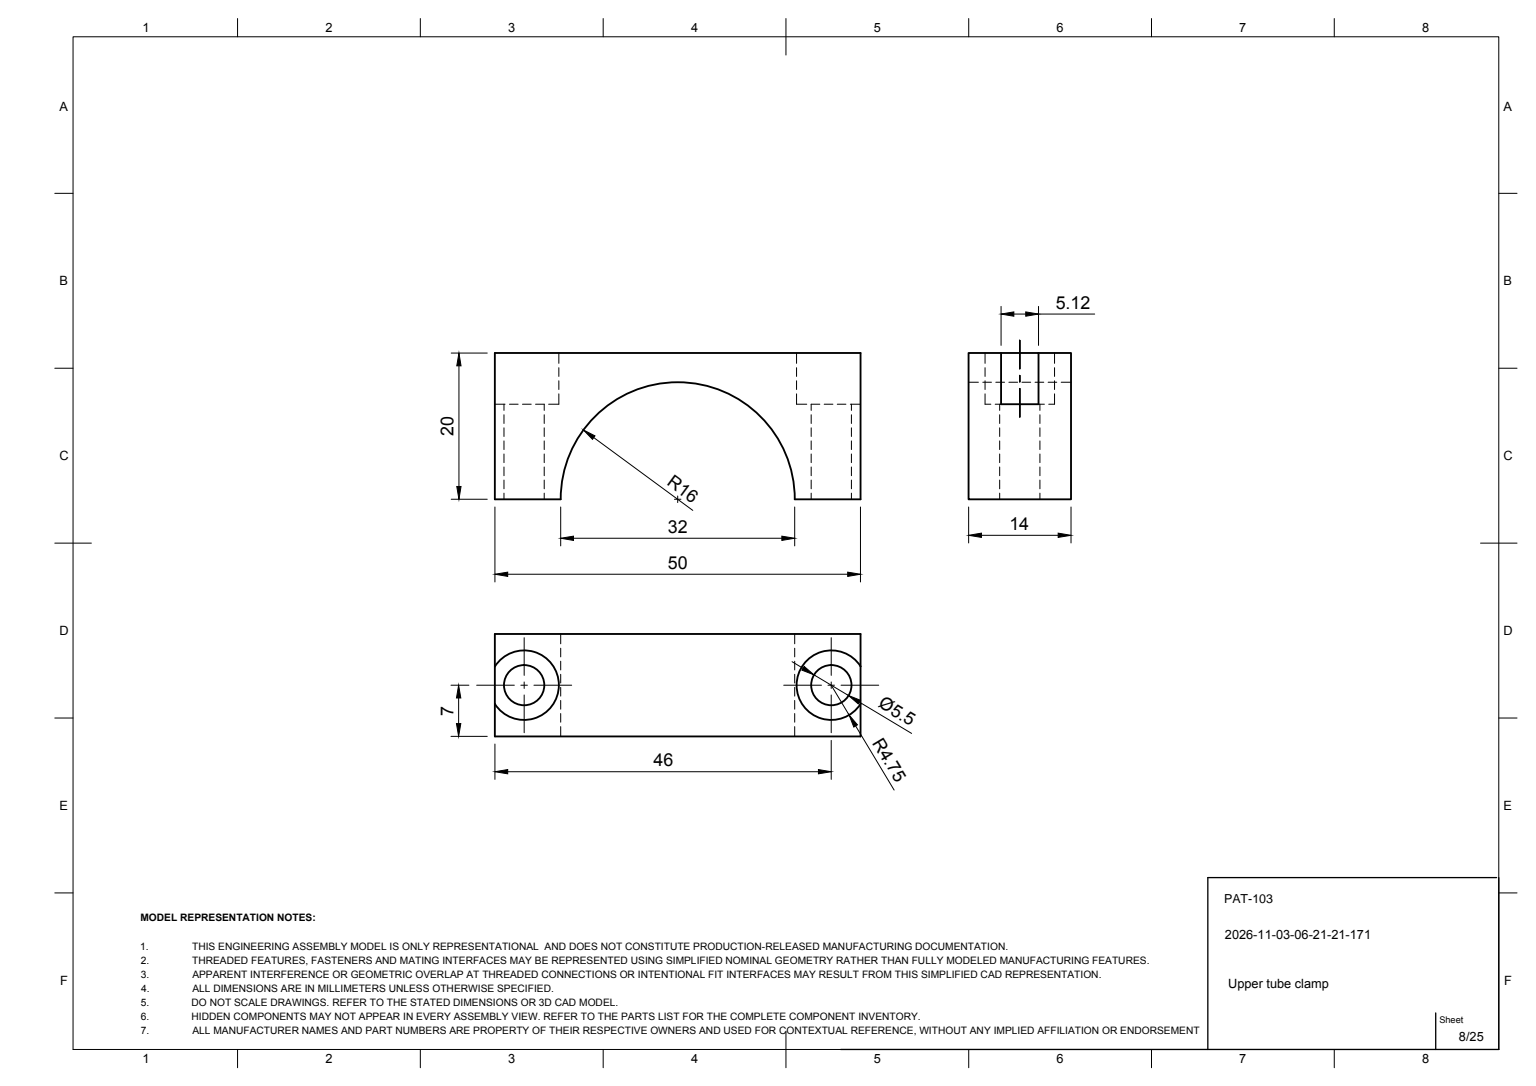
ISO-10303-21;
HEADER;
/* Generated by software containing ST-Developer
 * from STEP Tools, Inc. (www.steptools.com) 
 */

FILE_DESCRIPTION(
/* description */ ('Telescoping shaft support with lock collar'),
/* implementation_level */ '2;1');

FILE_NAME(
/* name */ 'Upper tube clamp.step',
/* time_stamp */ '2026-10-27T10:48:51-07:00',
/* author */ (''),
/* organization */ (''),
/* preprocessor_version */ 'ST-DEVELOPER v20.2',
/* originating_system */ 'Autodesk Translation Framework v15.17.0.0',
/* authorisation */ '');

FILE_SCHEMA (('AUTOMOTIVE_DESIGN { 1 0 10303 214 3 1 1 }'));
ENDSEC;

DATA;
#10=MECHANICAL_DESIGN_GEOMETRIC_PRESENTATION_REPRESENTATION('',(#244),#7349);
#204=SHAPE_REPRESENTATION_RELATIONSHIP('SRR','None',#7446,#224);
#224=ADVANCED_BREP_SHAPE_REPRESENTATION('',(#264),#7330);
#244=STYLED_ITEM('',(#7641),#264);
#264=MANIFOLD_SOLID_BREP('Body1',#3967);
#301=FACE_BOUND('',#790,.T.);
#302=FACE_BOUND('',#793,.T.);
#303=FACE_BOUND('',#802,.T.);
#304=FACE_BOUND('',#806,.T.);
#386=PLANE('',#4321);
#387=PLANE('',#4326);
#388=PLANE('',#4331);
#389=PLANE('',#4332);
#390=PLANE('',#4340);
#391=PLANE('',#4341);
#392=PLANE('',#4342);
#393=PLANE('',#4343);
#394=PLANE('',#4344);
#541=FACE_OUTER_BOUND('',#789,.T.);
#542=FACE_OUTER_BOUND('',#791,.T.);
#543=FACE_OUTER_BOUND('',#792,.T.);
#544=FACE_OUTER_BOUND('',#794,.T.);
#545=FACE_OUTER_BOUND('',#795,.T.);
#546=FACE_OUTER_BOUND('',#796,.T.);
#547=FACE_OUTER_BOUND('',#797,.T.);
#548=FACE_OUTER_BOUND('',#798,.T.);
#549=FACE_OUTER_BOUND('',#799,.T.);
#550=FACE_OUTER_BOUND('',#800,.T.);
#551=FACE_OUTER_BOUND('',#801,.T.);
#552=FACE_OUTER_BOUND('',#803,.T.);
#553=FACE_OUTER_BOUND('',#804,.T.);
#554=FACE_OUTER_BOUND('',#805,.T.);
#789=EDGE_LOOP('',(#2882,#2883));
#790=EDGE_LOOP('',(#2884));
#791=EDGE_LOOP('',(#2885,#2886,#2887,#2888));
#792=EDGE_LOOP('',(#2889,#2890));
#793=EDGE_LOOP('',(#2891));
#794=EDGE_LOOP('',(#2892,#2893,#2894,#2895));
#795=EDGE_LOOP('',(#2896,#2897,#2898,#2899,#2900,#2901,#2902,#2903));
#796=EDGE_LOOP('',(#2904,#2905,#2906,#2907,#2908,#2909,#2910,#2911));
#797=EDGE_LOOP('',(#2912,#2913,#2914,#2915));
#798=EDGE_LOOP('',(#2916,#2917,#2918,#2919));
#799=EDGE_LOOP('',(#2920,#2921,#2922,#2923));
#800=EDGE_LOOP('',(#2924,#2925,#2926,#2927,#2928,#2929));
#801=EDGE_LOOP('',(#2930,#2931,#2932,#2933));
#802=EDGE_LOOP('',(#2934));
#803=EDGE_LOOP('',(#2935,#2936,#2937,#2938,#2939,#2940));
#804=EDGE_LOOP('',(#2941,#2942,#2943,#2944,#2945,#2946,#2947,#2948));
#805=EDGE_LOOP('',(#2949,#2950,#2951,#2952));
#806=EDGE_LOOP('',(#2953));
#1085=LINE('',#6242,#1365);
#1086=LINE('',#6248,#1366);
#1087=LINE('',#6251,#1367);
#1088=LINE('',#6255,#1368);
#1089=LINE('',#6261,#1369);
#1090=LINE('',#6264,#1370);
#1091=LINE('',#6267,#1371);
#1092=LINE('',#6269,#1372);
#1093=LINE('',#6271,#1373);
#1094=LINE('',#6273,#1374);
#1095=LINE('',#6274,#1375);
#1096=LINE('',#6277,#1376);
#1097=LINE('',#6279,#1377);
#1098=LINE('',#6281,#1378);
#1099=LINE('',#6283,#1379);
#1100=LINE('',#6284,#1380);
#1101=LINE('',#6288,#1381);
#1102=LINE('',#6292,#1382);
#1103=LINE('',#6298,#1383);
#1104=LINE('',#6301,#1384);
#1105=LINE('',#6303,#1385);
#1106=LINE('',#6304,#1386);
#1107=LINE('',#6305,#1387);
#1108=LINE('',#6307,#1388);
#1109=LINE('',#6309,#1389);
#1110=LINE('',#6310,#1390);
#1365=VECTOR('',#4995,1.);
#1366=VECTOR('',#5002,1.);
#1367=VECTOR('',#5005,1.);
#1368=VECTOR('',#5008,1.);
#1369=VECTOR('',#5015,1.);
#1370=VECTOR('',#5018,1.);
#1371=VECTOR('',#5021,1.);
#1372=VECTOR('',#5022,1.);
#1373=VECTOR('',#5023,1.);
#1374=VECTOR('',#5024,1.);
#1375=VECTOR('',#5025,1.);
#1376=VECTOR('',#5028,1.);
#1377=VECTOR('',#5029,1.);
#1378=VECTOR('',#5030,1.);
#1379=VECTOR('',#5031,1.);
#1380=VECTOR('',#5032,1.);
#1381=VECTOR('',#5037,0.275);
#1382=VECTOR('',#5042,0.275);
#1383=VECTOR('',#5047,1.);
#1384=VECTOR('',#5050,1.);
#1385=VECTOR('',#5053,1.);
#1386=VECTOR('',#5054,1.);
#1387=VECTOR('',#5055,1.);
#1388=VECTOR('',#5058,1.);
#1389=VECTOR('',#5061,1.);
#1390=VECTOR('',#5062,1.);
#1649=CIRCLE('',#4322,0.475);
#1650=CIRCLE('',#4323,0.275);
#1651=CIRCLE('',#4325,0.475);
#1652=CIRCLE('',#4327,0.475);
#1653=CIRCLE('',#4328,0.275);
#1654=CIRCLE('',#4330,0.475);
#1655=CIRCLE('',#4334,0.275);
#1656=CIRCLE('',#4336,0.275);
#1657=CIRCLE('',#4338,1.6);
#1658=CIRCLE('',#4339,1.6);
#1878=VERTEX_POINT('',#6240);
#1879=VERTEX_POINT('',#6241);
#1880=VERTEX_POINT('',#6244);
#1881=VERTEX_POINT('',#6247);
#1882=VERTEX_POINT('',#6249);
#1883=VERTEX_POINT('',#6253);
#1884=VERTEX_POINT('',#6254);
#1885=VERTEX_POINT('',#6257);
#1886=VERTEX_POINT('',#6260);
#1887=VERTEX_POINT('',#6262);
#1888=VERTEX_POINT('',#6266);
#1889=VERTEX_POINT('',#6268);
#1890=VERTEX_POINT('',#6270);
#1891=VERTEX_POINT('',#6272);
#1892=VERTEX_POINT('',#6276);
#1893=VERTEX_POINT('',#6278);
#1894=VERTEX_POINT('',#6280);
#1895=VERTEX_POINT('',#6282);
#1896=VERTEX_POINT('',#6286);
#1897=VERTEX_POINT('',#6290);
#1898=VERTEX_POINT('',#6294);
#1899=VERTEX_POINT('',#6295);
#1900=VERTEX_POINT('',#6297);
#1901=VERTEX_POINT('',#6299);
#2253=EDGE_CURVE('',#1878,#1879,#1085,.T.);
#2254=EDGE_CURVE('',#1878,#1879,#1649,.T.);
#2255=EDGE_CURVE('',#1880,#1880,#1650,.T.);
#2256=EDGE_CURVE('',#1881,#1878,#1086,.T.);
#2257=EDGE_CURVE('',#1882,#1881,#1651,.T.);
#2258=EDGE_CURVE('',#1879,#1882,#1087,.T.);
#2259=EDGE_CURVE('',#1883,#1884,#1088,.T.);
#2260=EDGE_CURVE('',#1883,#1884,#1652,.T.);
#2261=EDGE_CURVE('',#1885,#1885,#1653,.T.);
#2262=EDGE_CURVE('',#1886,#1883,#1089,.T.);
#2263=EDGE_CURVE('',#1887,#1886,#1654,.T.);
#2264=EDGE_CURVE('',#1884,#1887,#1090,.T.);
#2265=EDGE_CURVE('',#1888,#1882,#1091,.T.);
#2266=EDGE_CURVE('',#1889,#1888,#1092,.T.);
#2267=EDGE_CURVE('',#1889,#1890,#1093,.T.);
#2268=EDGE_CURVE('',#1890,#1891,#1094,.T.);
#2269=EDGE_CURVE('',#1881,#1891,#1095,.T.);
#2270=EDGE_CURVE('',#1892,#1887,#1096,.T.);
#2271=EDGE_CURVE('',#1893,#1892,#1097,.T.);
#2272=EDGE_CURVE('',#1893,#1894,#1098,.T.);
#2273=EDGE_CURVE('',#1894,#1895,#1099,.T.);
#2274=EDGE_CURVE('',#1886,#1895,#1100,.T.);
#2275=EDGE_CURVE('',#1896,#1896,#1655,.T.);
#2276=EDGE_CURVE('',#1896,#1880,#1101,.T.);
#2277=EDGE_CURVE('',#1897,#1897,#1656,.T.);
#2278=EDGE_CURVE('',#1897,#1885,#1102,.T.);
#2279=EDGE_CURVE('',#1898,#1899,#1657,.T.);
#2280=EDGE_CURVE('',#1900,#1898,#1103,.T.);
#2281=EDGE_CURVE('',#1901,#1900,#1658,.T.);
#2282=EDGE_CURVE('',#1899,#1901,#1104,.T.);
#2283=EDGE_CURVE('',#1900,#1893,#1105,.T.);
#2284=EDGE_CURVE('',#1891,#1892,#1106,.T.);
#2285=EDGE_CURVE('',#1890,#1901,#1107,.T.);
#2286=EDGE_CURVE('',#1894,#1898,#1108,.T.);
#2287=EDGE_CURVE('',#1899,#1889,#1109,.T.);
#2288=EDGE_CURVE('',#1895,#1888,#1110,.T.);
#2882=ORIENTED_EDGE('',*,*,#2253,.F.);
#2883=ORIENTED_EDGE('',*,*,#2254,.T.);
#2884=ORIENTED_EDGE('',*,*,#2255,.F.);
#2885=ORIENTED_EDGE('',*,*,#2256,.F.);
#2886=ORIENTED_EDGE('',*,*,#2257,.F.);
#2887=ORIENTED_EDGE('',*,*,#2258,.F.);
#2888=ORIENTED_EDGE('',*,*,#2254,.F.);
#2889=ORIENTED_EDGE('',*,*,#2259,.F.);
#2890=ORIENTED_EDGE('',*,*,#2260,.T.);
#2891=ORIENTED_EDGE('',*,*,#2261,.F.);
#2892=ORIENTED_EDGE('',*,*,#2262,.F.);
#2893=ORIENTED_EDGE('',*,*,#2263,.F.);
#2894=ORIENTED_EDGE('',*,*,#2264,.F.);
#2895=ORIENTED_EDGE('',*,*,#2260,.F.);
#2896=ORIENTED_EDGE('',*,*,#2256,.T.);
#2897=ORIENTED_EDGE('',*,*,#2253,.T.);
#2898=ORIENTED_EDGE('',*,*,#2258,.T.);
#2899=ORIENTED_EDGE('',*,*,#2265,.F.);
#2900=ORIENTED_EDGE('',*,*,#2266,.F.);
#2901=ORIENTED_EDGE('',*,*,#2267,.T.);
#2902=ORIENTED_EDGE('',*,*,#2268,.T.);
#2903=ORIENTED_EDGE('',*,*,#2269,.F.);
#2904=ORIENTED_EDGE('',*,*,#2262,.T.);
#2905=ORIENTED_EDGE('',*,*,#2259,.T.);
#2906=ORIENTED_EDGE('',*,*,#2264,.T.);
#2907=ORIENTED_EDGE('',*,*,#2270,.F.);
#2908=ORIENTED_EDGE('',*,*,#2271,.F.);
#2909=ORIENTED_EDGE('',*,*,#2272,.T.);
#2910=ORIENTED_EDGE('',*,*,#2273,.T.);
#2911=ORIENTED_EDGE('',*,*,#2274,.F.);
#2912=ORIENTED_EDGE('',*,*,#2275,.F.);
#2913=ORIENTED_EDGE('',*,*,#2276,.T.);
#2914=ORIENTED_EDGE('',*,*,#2255,.T.);
#2915=ORIENTED_EDGE('',*,*,#2276,.F.);
#2916=ORIENTED_EDGE('',*,*,#2277,.F.);
#2917=ORIENTED_EDGE('',*,*,#2278,.T.);
#2918=ORIENTED_EDGE('',*,*,#2261,.T.);
#2919=ORIENTED_EDGE('',*,*,#2278,.F.);
#2920=ORIENTED_EDGE('',*,*,#2279,.F.);
#2921=ORIENTED_EDGE('',*,*,#2280,.F.);
#2922=ORIENTED_EDGE('',*,*,#2281,.F.);
#2923=ORIENTED_EDGE('',*,*,#2282,.F.);
#2924=ORIENTED_EDGE('',*,*,#2281,.T.);
#2925=ORIENTED_EDGE('',*,*,#2283,.T.);
#2926=ORIENTED_EDGE('',*,*,#2271,.T.);
#2927=ORIENTED_EDGE('',*,*,#2284,.F.);
#2928=ORIENTED_EDGE('',*,*,#2268,.F.);
#2929=ORIENTED_EDGE('',*,*,#2285,.T.);
#2930=ORIENTED_EDGE('',*,*,#2280,.T.);
#2931=ORIENTED_EDGE('',*,*,#2286,.F.);
#2932=ORIENTED_EDGE('',*,*,#2272,.F.);
#2933=ORIENTED_EDGE('',*,*,#2283,.F.);
#2934=ORIENTED_EDGE('',*,*,#2277,.T.);
#2935=ORIENTED_EDGE('',*,*,#2279,.T.);
#2936=ORIENTED_EDGE('',*,*,#2287,.T.);
#2937=ORIENTED_EDGE('',*,*,#2266,.T.);
#2938=ORIENTED_EDGE('',*,*,#2288,.F.);
#2939=ORIENTED_EDGE('',*,*,#2273,.F.);
#2940=ORIENTED_EDGE('',*,*,#2286,.T.);
#2941=ORIENTED_EDGE('',*,*,#2257,.T.);
#2942=ORIENTED_EDGE('',*,*,#2269,.T.);
#2943=ORIENTED_EDGE('',*,*,#2284,.T.);
#2944=ORIENTED_EDGE('',*,*,#2270,.T.);
#2945=ORIENTED_EDGE('',*,*,#2263,.T.);
#2946=ORIENTED_EDGE('',*,*,#2274,.T.);
#2947=ORIENTED_EDGE('',*,*,#2288,.T.);
#2948=ORIENTED_EDGE('',*,*,#2265,.T.);
#2949=ORIENTED_EDGE('',*,*,#2282,.T.);
#2950=ORIENTED_EDGE('',*,*,#2285,.F.);
#2951=ORIENTED_EDGE('',*,*,#2267,.F.);
#2952=ORIENTED_EDGE('',*,*,#2287,.F.);
#2953=ORIENTED_EDGE('',*,*,#2275,.T.);
#3679=CYLINDRICAL_SURFACE('',#4324,0.475);
#3680=CYLINDRICAL_SURFACE('',#4329,0.475);
#3681=CYLINDRICAL_SURFACE('',#4333,0.275);
#3682=CYLINDRICAL_SURFACE('',#4335,0.275);
#3683=CYLINDRICAL_SURFACE('',#4337,1.6);
#3784=ADVANCED_FACE('',(#541,#301),#386,.T.);
#3785=ADVANCED_FACE('',(#542),#3679,.F.);
#3786=ADVANCED_FACE('',(#543,#302),#387,.T.);
#3787=ADVANCED_FACE('',(#544),#3680,.F.);
#3788=ADVANCED_FACE('',(#545),#388,.T.);
#3789=ADVANCED_FACE('',(#546),#389,.T.);
#3790=ADVANCED_FACE('',(#547),#3681,.F.);
#3791=ADVANCED_FACE('',(#548),#3682,.F.);
#3792=ADVANCED_FACE('',(#549),#3683,.F.);
#3793=ADVANCED_FACE('',(#550),#390,.T.);
#3794=ADVANCED_FACE('',(#551,#303),#391,.F.);
#3795=ADVANCED_FACE('',(#552),#392,.T.);
#3796=ADVANCED_FACE('',(#553),#393,.T.);
#3797=ADVANCED_FACE('',(#554,#304),#394,.F.);
#3967=CLOSED_SHELL('',(#3784,#3785,#3786,#3787,#3788,#3789,#3790,#3791,
#3792,#3793,#3794,#3795,#3796,#3797));
#4320=AXIS2_PLACEMENT_3D('',#6238,#4991,#4992);
#4321=AXIS2_PLACEMENT_3D('',#6239,#4993,#4994);
#4322=AXIS2_PLACEMENT_3D('',#6243,#4996,#4997);
#4323=AXIS2_PLACEMENT_3D('',#6245,#4998,#4999);
#4324=AXIS2_PLACEMENT_3D('',#6246,#5000,#5001);
#4325=AXIS2_PLACEMENT_3D('',#6250,#5003,#5004);
#4326=AXIS2_PLACEMENT_3D('',#6252,#5006,#5007);
#4327=AXIS2_PLACEMENT_3D('',#6256,#5009,#5010);
#4328=AXIS2_PLACEMENT_3D('',#6258,#5011,#5012);
#4329=AXIS2_PLACEMENT_3D('',#6259,#5013,#5014);
#4330=AXIS2_PLACEMENT_3D('',#6263,#5016,#5017);
#4331=AXIS2_PLACEMENT_3D('',#6265,#5019,#5020);
#4332=AXIS2_PLACEMENT_3D('',#6275,#5026,#5027);
#4333=AXIS2_PLACEMENT_3D('',#6285,#5033,#5034);
#4334=AXIS2_PLACEMENT_3D('',#6287,#5035,#5036);
#4335=AXIS2_PLACEMENT_3D('',#6289,#5038,#5039);
#4336=AXIS2_PLACEMENT_3D('',#6291,#5040,#5041);
#4337=AXIS2_PLACEMENT_3D('',#6293,#5043,#5044);
#4338=AXIS2_PLACEMENT_3D('',#6296,#5045,#5046);
#4339=AXIS2_PLACEMENT_3D('',#6300,#5048,#5049);
#4340=AXIS2_PLACEMENT_3D('',#6302,#5051,#5052);
#4341=AXIS2_PLACEMENT_3D('',#6306,#5056,#5057);
#4342=AXIS2_PLACEMENT_3D('',#6308,#5059,#5060);
#4343=AXIS2_PLACEMENT_3D('',#6311,#5063,#5064);
#4344=AXIS2_PLACEMENT_3D('',#6312,#5065,#5066);
#4991=DIRECTION('axis',(0.,0.,1.));
#4992=DIRECTION('refdir',(1.,0.,0.));
#4993=DIRECTION('center_axis',(0.,0.,1.));
#4994=DIRECTION('ref_axis',(1.,0.,0.));
#4995=DIRECTION('',(-1.,0.,0.));
#4996=DIRECTION('center_axis',(0.,0.,1.));
#4997=DIRECTION('ref_axis',(1.,0.,0.));
#4998=DIRECTION('center_axis',(0.,0.,1.));
#4999=DIRECTION('ref_axis',(1.,0.,0.));
#5000=DIRECTION('center_axis',(0.,0.,1.));
#5001=DIRECTION('ref_axis',(2.83276944882399E-16,1.,0.));
#5002=DIRECTION('',(0.,0.,-1.));
#5003=DIRECTION('center_axis',(0.,0.,-1.));
#5004=DIRECTION('ref_axis',(1.,0.,0.));
#5005=DIRECTION('',(0.,0.,1.));
#5006=DIRECTION('center_axis',(0.,0.,1.));
#5007=DIRECTION('ref_axis',(1.,0.,0.));
#5008=DIRECTION('',(1.,0.,0.));
#5009=DIRECTION('center_axis',(0.,0.,1.));
#5010=DIRECTION('ref_axis',(1.,0.,0.));
#5011=DIRECTION('center_axis',(0.,0.,1.));
#5012=DIRECTION('ref_axis',(1.,0.,0.));
#5013=DIRECTION('center_axis',(0.,0.,1.));
#5014=DIRECTION('ref_axis',(-1.83697019872103E-16,-1.,0.));
#5015=DIRECTION('',(0.,0.,-1.));
#5016=DIRECTION('center_axis',(0.,0.,-1.));
#5017=DIRECTION('ref_axis',(1.,0.,0.));
#5018=DIRECTION('',(0.,0.,1.));
#5019=DIRECTION('center_axis',(0.,-1.,0.));
#5020=DIRECTION('ref_axis',(1.,0.,0.));
#5021=DIRECTION('',(1.,0.,0.));
#5022=DIRECTION('',(0.,0.,1.));
#5023=DIRECTION('',(1.,0.,0.));
#5024=DIRECTION('',(0.,0.,1.));
#5025=DIRECTION('',(1.,0.,0.));
#5026=DIRECTION('center_axis',(0.,1.,0.));
#5027=DIRECTION('ref_axis',(-1.,0.,0.));
#5028=DIRECTION('',(-1.,0.,0.));
#5029=DIRECTION('',(0.,0.,1.));
#5030=DIRECTION('',(-1.,0.,0.));
#5031=DIRECTION('',(0.,0.,1.));
#5032=DIRECTION('',(-1.,0.,0.));
#5033=DIRECTION('center_axis',(0.,0.,1.));
#5034=DIRECTION('ref_axis',(1.,0.,0.));
#5035=DIRECTION('center_axis',(0.,0.,1.));
#5036=DIRECTION('ref_axis',(1.,0.,0.));
#5037=DIRECTION('',(0.,0.,1.));
#5038=DIRECTION('center_axis',(0.,0.,1.));
#5039=DIRECTION('ref_axis',(1.,0.,0.));
#5040=DIRECTION('center_axis',(0.,0.,1.));
#5041=DIRECTION('ref_axis',(1.,0.,0.));
#5042=DIRECTION('',(0.,0.,1.));
#5043=DIRECTION('center_axis',(1.,0.,0.));
#5044=DIRECTION('ref_axis',(0.,1.22464679914735E-16,1.));
#5045=DIRECTION('center_axis',(1.,0.,0.));
#5046=DIRECTION('ref_axis',(0.,0.,-1.));
#5047=DIRECTION('',(-1.,0.,0.));
#5048=DIRECTION('center_axis',(-1.,0.,0.));
#5049=DIRECTION('ref_axis',(0.,0.,-1.));
#5050=DIRECTION('',(1.,0.,0.));
#5051=DIRECTION('center_axis',(1.,0.,0.));
#5052=DIRECTION('ref_axis',(0.,1.,0.));
#5053=DIRECTION('',(0.,1.,0.));
#5054=DIRECTION('',(0.,1.,0.));
#5055=DIRECTION('',(0.,1.,0.));
#5056=DIRECTION('center_axis',(0.,0.,1.));
#5057=DIRECTION('ref_axis',(1.,0.,0.));
#5058=DIRECTION('',(0.,-1.,0.));
#5059=DIRECTION('center_axis',(-1.,0.,0.));
#5060=DIRECTION('ref_axis',(0.,-1.,0.));
#5061=DIRECTION('',(0.,-1.,0.));
#5062=DIRECTION('',(0.,-1.,0.));
#5063=DIRECTION('center_axis',(0.,0.,1.));
#5064=DIRECTION('ref_axis',(1.,0.,0.));
#5065=DIRECTION('center_axis',(0.,0.,1.));
#5066=DIRECTION('ref_axis',(1.,0.,0.));
#6238=CARTESIAN_POINT('',(0.,0.,0.));
#6239=CARTESIAN_POINT('Origin',(2.2,-2.1,4.8));
#6240=CARTESIAN_POINT('',(2.45617376914899,-2.5,4.8));
#6241=CARTESIAN_POINT('',(1.94382623085101,-2.5,4.8));
#6242=CARTESIAN_POINT('',(1.85,-2.5,4.8));
#6243=CARTESIAN_POINT('Origin',(2.2,-2.1,4.8));
#6244=CARTESIAN_POINT('',(1.925,-2.1,4.8));
#6245=CARTESIAN_POINT('Origin',(2.2,-2.1,4.8));
#6246=CARTESIAN_POINT('Origin',(2.2,-2.1,4.8));
#6247=CARTESIAN_POINT('',(2.45617376914899,-2.5,5.5));
#6248=CARTESIAN_POINT('',(2.45617376914899,-2.5,4.8));
#6249=CARTESIAN_POINT('',(1.94382623085101,-2.5,5.5));
#6250=CARTESIAN_POINT('Origin',(2.2,-2.1,5.5));
#6251=CARTESIAN_POINT('',(1.94382623085101,-2.5,4.8));
#6252=CARTESIAN_POINT('Origin',(2.2,2.1,4.8));
#6253=CARTESIAN_POINT('',(1.94382623085101,2.5,4.8));
#6254=CARTESIAN_POINT('',(2.45617376914899,2.5,4.8));
#6255=CARTESIAN_POINT('',(2.55,2.5,4.8));
#6256=CARTESIAN_POINT('Origin',(2.2,2.1,4.8));
#6257=CARTESIAN_POINT('',(1.925,2.1,4.8));
#6258=CARTESIAN_POINT('Origin',(2.2,2.1,4.8));
#6259=CARTESIAN_POINT('Origin',(2.2,2.1,4.8));
#6260=CARTESIAN_POINT('',(1.94382623085101,2.5,5.5));
#6261=CARTESIAN_POINT('',(1.94382623085101,2.5,4.8));
#6262=CARTESIAN_POINT('',(2.45617376914899,2.5,5.5));
#6263=CARTESIAN_POINT('Origin',(2.2,2.1,5.5));
#6264=CARTESIAN_POINT('',(2.45617376914899,2.5,4.8));
#6265=CARTESIAN_POINT('Origin',(1.5,-2.5,3.5));
#6266=CARTESIAN_POINT('',(1.5,-2.5,5.5));
#6267=CARTESIAN_POINT('',(1.5,-2.5,5.5));
#6268=CARTESIAN_POINT('',(1.5,-2.5,3.5));
#6269=CARTESIAN_POINT('',(1.5,-2.5,3.5));
#6270=CARTESIAN_POINT('',(2.9,-2.5,3.5));
#6271=CARTESIAN_POINT('',(1.5,-2.5,3.5));
#6272=CARTESIAN_POINT('',(2.9,-2.5,5.5));
#6273=CARTESIAN_POINT('',(2.9,-2.5,3.5));
#6274=CARTESIAN_POINT('',(1.5,-2.5,5.5));
#6275=CARTESIAN_POINT('Origin',(2.9,2.5,3.5));
#6276=CARTESIAN_POINT('',(2.9,2.5,5.5));
#6277=CARTESIAN_POINT('',(2.9,2.5,5.5));
#6278=CARTESIAN_POINT('',(2.9,2.5,3.5));
#6279=CARTESIAN_POINT('',(2.9,2.5,3.5));
#6280=CARTESIAN_POINT('',(1.5,2.5,3.5));
#6281=CARTESIAN_POINT('',(2.9,2.5,3.5));
#6282=CARTESIAN_POINT('',(1.5,2.5,5.5));
#6283=CARTESIAN_POINT('',(1.5,2.5,3.5));
#6284=CARTESIAN_POINT('',(2.9,2.5,5.5));
#6285=CARTESIAN_POINT('Origin',(2.2,-2.1,3.4));
#6286=CARTESIAN_POINT('',(1.925,-2.1,3.5));
#6287=CARTESIAN_POINT('Origin',(2.2,-2.1,3.5));
#6288=CARTESIAN_POINT('',(1.925,-2.1,3.4));
#6289=CARTESIAN_POINT('Origin',(2.2,2.1,3.4));
#6290=CARTESIAN_POINT('',(1.925,2.1,3.5));
#6291=CARTESIAN_POINT('Origin',(2.2,2.1,3.5));
#6292=CARTESIAN_POINT('',(1.925,2.1,3.4));
#6293=CARTESIAN_POINT('Origin',(1.4,0.,3.5));
#6294=CARTESIAN_POINT('',(1.5,1.6,3.5));
#6295=CARTESIAN_POINT('',(1.5,-1.6,3.5));
#6296=CARTESIAN_POINT('Origin',(1.5,0.,3.5));
#6297=CARTESIAN_POINT('',(2.9,1.6,3.5));
#6298=CARTESIAN_POINT('',(1.4,1.6,3.5));
#6299=CARTESIAN_POINT('',(2.9,-1.6,3.5));
#6300=CARTESIAN_POINT('Origin',(2.9,0.,3.5));
#6301=CARTESIAN_POINT('',(1.4,-1.6,3.5));
#6302=CARTESIAN_POINT('Origin',(2.9,-2.5,3.5));
#6303=CARTESIAN_POINT('',(2.9,-2.5,3.5));
#6304=CARTESIAN_POINT('',(2.9,-2.5,5.5));
#6305=CARTESIAN_POINT('',(2.9,-2.5,3.5));
#6306=CARTESIAN_POINT('Origin',(2.2,0.,3.5));
#6307=CARTESIAN_POINT('',(1.5,2.5,3.5));
#6308=CARTESIAN_POINT('Origin',(1.5,2.5,3.5));
#6309=CARTESIAN_POINT('',(1.5,2.5,3.5));
#6310=CARTESIAN_POINT('',(1.5,2.5,5.5));
#6311=CARTESIAN_POINT('Origin',(2.2,0.,5.5));
#6312=CARTESIAN_POINT('Origin',(2.2,0.,3.5));
#7305=UNCERTAINTY_MEASURE_WITH_UNIT(LENGTH_MEASURE(0.001),#7350,
'DISTANCE_ACCURACY_VALUE',
'Maximum model space distance between geometric entities at asserted c
onnectivities');
#7324=UNCERTAINTY_MEASURE_WITH_UNIT(LENGTH_MEASURE(0.001),#7350,
'DISTANCE_ACCURACY_VALUE',
'Maximum model space distance between geometric entities at asserted c
onnectivities');
#7330=(
GEOMETRIC_REPRESENTATION_CONTEXT(3)
GLOBAL_UNCERTAINTY_ASSIGNED_CONTEXT((#7305))
GLOBAL_UNIT_ASSIGNED_CONTEXT((#7350,#7352,#7353))
REPRESENTATION_CONTEXT('','3D')
);
#7349=(
GEOMETRIC_REPRESENTATION_CONTEXT(3)
GLOBAL_UNCERTAINTY_ASSIGNED_CONTEXT((#7324))
GLOBAL_UNIT_ASSIGNED_CONTEXT((#7350,#7352,#7353))
REPRESENTATION_CONTEXT('','3D')
);
#7350=(
LENGTH_UNIT()
NAMED_UNIT(*)
SI_UNIT(.CENTI.,.METRE.)
);
#7352=(
NAMED_UNIT(*)
PLANE_ANGLE_UNIT()
SI_UNIT($,.RADIAN.)
);
#7353=(
NAMED_UNIT(*)
SI_UNIT($,.STERADIAN.)
SOLID_ANGLE_UNIT()
);
#7359=SHAPE_DEFINITION_REPRESENTATION(#7383,#7446);
#7383=PRODUCT_DEFINITION_SHAPE('',$,#7471);
#7446=SHAPE_REPRESENTATION('',(#4320),#7330);
#7465=PRODUCT_DEFINITION_CONTEXT('part definition',#7539,'design');
#7471=PRODUCT_DEFINITION('Upper tube clamp','Upper tube clamp',#7495,#7465);
#7495=PRODUCT_DEFINITION_FORMATION('',$,#7546);
#7539=APPLICATION_CONTEXT(
'Core Data for Automotive Mechanical Design Process');
#7540=PRODUCT_CONTEXT('part definition',#7539,'mechanical');
#7546=PRODUCT('Upper tube clamp','Upper tube clamp','Upper tube clamp',
(#7540));
#7635=COLOUR_RGB('Off White',0.89,0.88,0.83);
#7636=FILL_AREA_STYLE_COLOUR('',#7635);
#7637=FILL_AREA_STYLE('',(#7636));
#7638=SURFACE_STYLE_FILL_AREA(#7637);
#7639=SURFACE_SIDE_STYLE('',(#7638));
#7640=SURFACE_STYLE_USAGE(.BOTH.,#7639);
#7641=PRESENTATION_STYLE_ASSIGNMENT((#7640));
ENDSEC;
END-ISO-10303-21;
